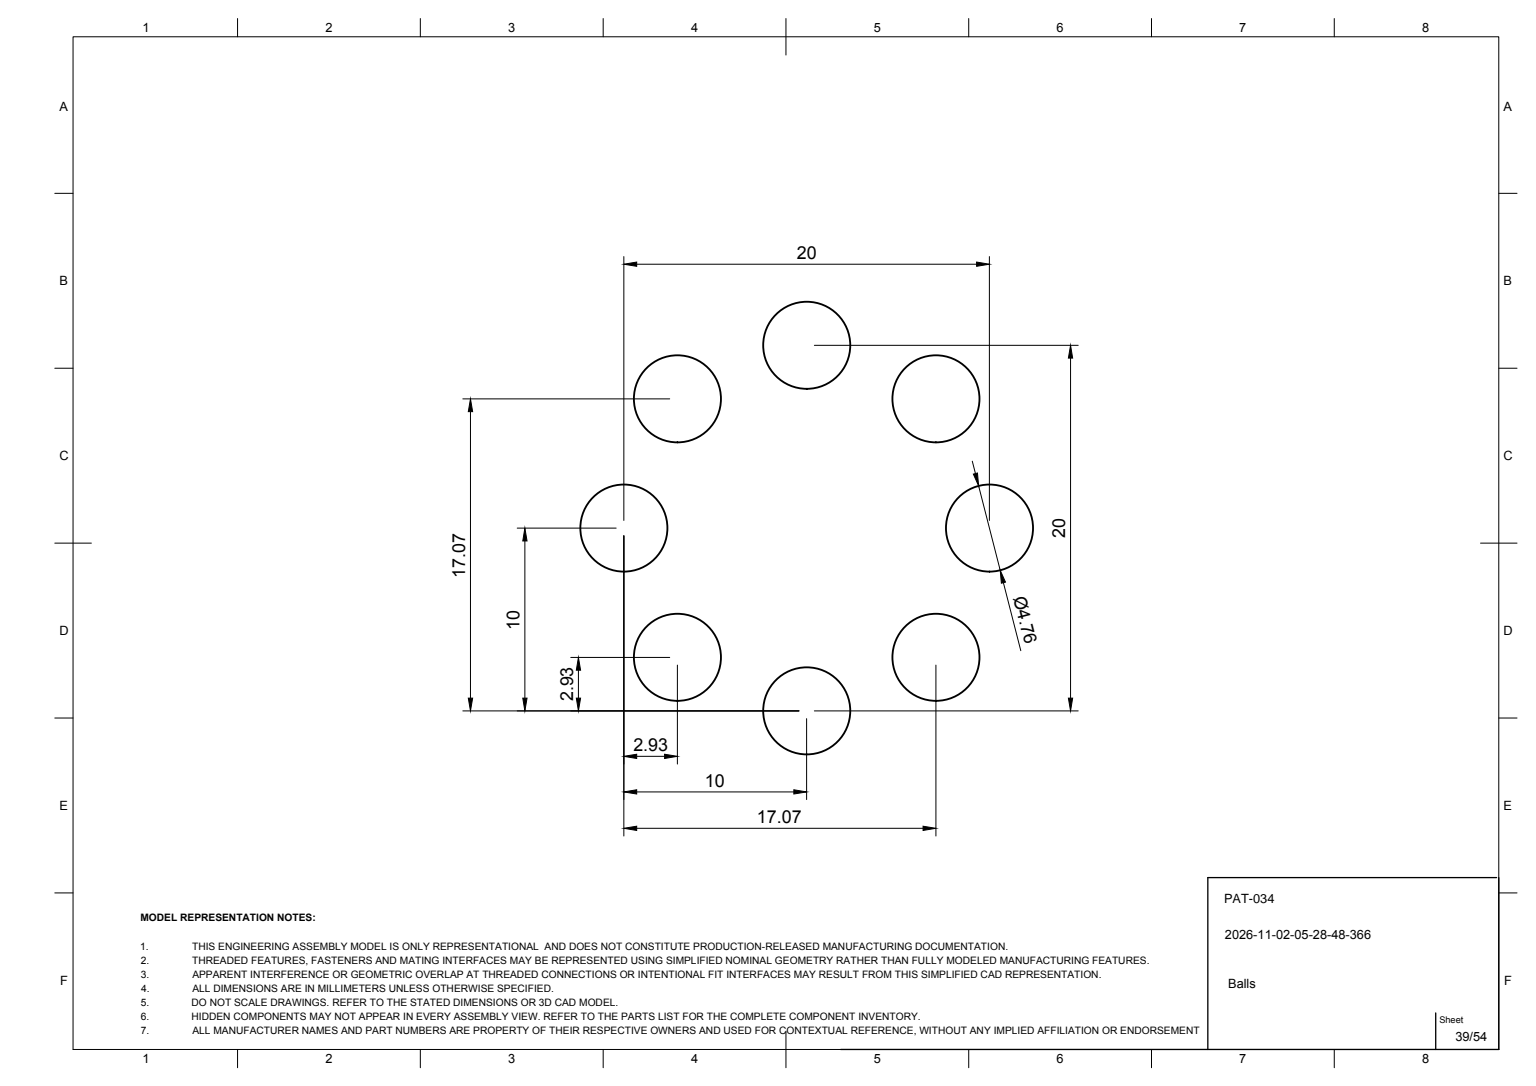
ISO-10303-21;
HEADER;
/* Generated by software containing ST-Developer
 * from STEP Tools, Inc. (www.steptools.com) 
 */

FILE_DESCRIPTION(
/* description */ ('Fatigue rig crank-slider'),
/* implementation_level */ '2;1');

FILE_NAME(
/* name */ 'Balls.step',
/* time_stamp */ '2026-10-28T03:24:50-07:00',
/* author */ (''),
/* organization */ (''),
/* preprocessor_version */ 'ST-DEVELOPER v20.2',
/* originating_system */ 'Autodesk Translation Framework v15.17.0.0',
/* authorisation */ '');

FILE_SCHEMA (('AUTOMOTIVE_DESIGN { 1 0 10303 214 3 1 1 }'));
ENDSEC;

DATA;
#10=MECHANICAL_DESIGN_GEOMETRIC_PRESENTATION_REPRESENTATION('',(#622,#623,#624,#625,#626,#627,#628,#629),#16911);
#471=SPHERICAL_SURFACE('',#10148,0.23815);
#472=SPHERICAL_SURFACE('',#10150,0.23815);
#473=SPHERICAL_SURFACE('',#10152,0.23815);
#474=SPHERICAL_SURFACE('',#10154,0.23815);
#475=SPHERICAL_SURFACE('',#10156,0.23815);
#476=SPHERICAL_SURFACE('',#10158,0.23815);
#477=SPHERICAL_SURFACE('',#10160,0.23815);
#478=SPHERICAL_SURFACE('',#10162,0.23815);
#521=SHAPE_REPRESENTATION_RELATIONSHIP('SRR','None',#17164,#571);
#571=ADVANCED_BREP_SHAPE_REPRESENTATION('',(#679,#680,#681,#682,#683,#684,
#685,#686),#16893);
#622=STYLED_ITEM('',(#17487),#679);
#623=STYLED_ITEM('',(#17487),#680);
#624=STYLED_ITEM('',(#17487),#681);
#625=STYLED_ITEM('',(#17487),#682);
#626=STYLED_ITEM('',(#17487),#683);
#627=STYLED_ITEM('',(#17487),#684);
#628=STYLED_ITEM('',(#17487),#685);
#629=STYLED_ITEM('',(#17487),#686);
#679=MANIFOLD_SOLID_BREP('Body1',#8915);
#680=MANIFOLD_SOLID_BREP('Body2',#8916);
#681=MANIFOLD_SOLID_BREP('Body3',#8917);
#682=MANIFOLD_SOLID_BREP('Body4',#8918);
#683=MANIFOLD_SOLID_BREP('Body5',#8919);
#684=MANIFOLD_SOLID_BREP('Body6',#8920);
#685=MANIFOLD_SOLID_BREP('Body7',#8921);
#686=MANIFOLD_SOLID_BREP('Body8',#8922);
#1558=FACE_OUTER_BOUND('',#2239,.T.);
#1559=FACE_OUTER_BOUND('',#2240,.T.);
#1560=FACE_OUTER_BOUND('',#2241,.T.);
#1561=FACE_OUTER_BOUND('',#2242,.T.);
#1562=FACE_OUTER_BOUND('',#2243,.T.);
#1563=FACE_OUTER_BOUND('',#2244,.T.);
#1564=FACE_OUTER_BOUND('',#2245,.T.);
#1565=FACE_OUTER_BOUND('',#2246,.T.);
#2239=EDGE_LOOP('',(#7404,#7405));
#2240=EDGE_LOOP('',(#7406,#7407));
#2241=EDGE_LOOP('',(#7408,#7409));
#2242=EDGE_LOOP('',(#7410,#7411));
#2243=EDGE_LOOP('',(#7412,#7413));
#2244=EDGE_LOOP('',(#7414,#7415));
#2245=EDGE_LOOP('',(#7416,#7417));
#2246=EDGE_LOOP('',(#7418,#7419));
#4023=CIRCLE('',#10149,0.23815);
#4024=CIRCLE('',#10151,0.23815);
#4025=CIRCLE('',#10153,0.23815);
#4026=CIRCLE('',#10155,0.23815);
#4027=CIRCLE('',#10157,0.23815);
#4028=CIRCLE('',#10159,0.23815);
#4029=CIRCLE('',#10161,0.23815);
#4030=CIRCLE('',#10163,0.23815);
#4625=VERTEX_POINT('',#15501);
#4626=VERTEX_POINT('',#15502);
#4627=VERTEX_POINT('',#15505);
#4628=VERTEX_POINT('',#15506);
#4629=VERTEX_POINT('',#15509);
#4630=VERTEX_POINT('',#15510);
#4631=VERTEX_POINT('',#15513);
#4632=VERTEX_POINT('',#15514);
#4633=VERTEX_POINT('',#15517);
#4634=VERTEX_POINT('',#15518);
#4635=VERTEX_POINT('',#15521);
#4636=VERTEX_POINT('',#15522);
#4637=VERTEX_POINT('',#15525);
#4638=VERTEX_POINT('',#15526);
#4639=VERTEX_POINT('',#15529);
#4640=VERTEX_POINT('',#15530);
#5600=EDGE_CURVE('',#4625,#4626,#4023,.T.);
#5601=EDGE_CURVE('',#4627,#4628,#4024,.T.);
#5602=EDGE_CURVE('',#4629,#4630,#4025,.T.);
#5603=EDGE_CURVE('',#4631,#4632,#4026,.T.);
#5604=EDGE_CURVE('',#4633,#4634,#4027,.T.);
#5605=EDGE_CURVE('',#4635,#4636,#4028,.T.);
#5606=EDGE_CURVE('',#4637,#4638,#4029,.T.);
#5607=EDGE_CURVE('',#4639,#4640,#4030,.T.);
#7404=ORIENTED_EDGE('',*,*,#5600,.T.);
#7405=ORIENTED_EDGE('',*,*,#5600,.F.);
#7406=ORIENTED_EDGE('',*,*,#5601,.T.);
#7407=ORIENTED_EDGE('',*,*,#5601,.F.);
#7408=ORIENTED_EDGE('',*,*,#5602,.T.);
#7409=ORIENTED_EDGE('',*,*,#5602,.F.);
#7410=ORIENTED_EDGE('',*,*,#5603,.T.);
#7411=ORIENTED_EDGE('',*,*,#5603,.F.);
#7412=ORIENTED_EDGE('',*,*,#5604,.T.);
#7413=ORIENTED_EDGE('',*,*,#5604,.F.);
#7414=ORIENTED_EDGE('',*,*,#5605,.T.);
#7415=ORIENTED_EDGE('',*,*,#5605,.F.);
#7416=ORIENTED_EDGE('',*,*,#5606,.T.);
#7417=ORIENTED_EDGE('',*,*,#5606,.F.);
#7418=ORIENTED_EDGE('',*,*,#5607,.T.);
#7419=ORIENTED_EDGE('',*,*,#5607,.F.);
#8696=ADVANCED_FACE('',(#1558),#471,.T.);
#8697=ADVANCED_FACE('',(#1559),#472,.T.);
#8698=ADVANCED_FACE('',(#1560),#473,.T.);
#8699=ADVANCED_FACE('',(#1561),#474,.T.);
#8700=ADVANCED_FACE('',(#1562),#475,.T.);
#8701=ADVANCED_FACE('',(#1563),#476,.T.);
#8702=ADVANCED_FACE('',(#1564),#477,.T.);
#8703=ADVANCED_FACE('',(#1565),#478,.T.);
#8915=CLOSED_SHELL('',(#8696));
#8916=CLOSED_SHELL('',(#8697));
#8917=CLOSED_SHELL('',(#8698));
#8918=CLOSED_SHELL('',(#8699));
#8919=CLOSED_SHELL('',(#8700));
#8920=CLOSED_SHELL('',(#8701));
#8921=CLOSED_SHELL('',(#8702));
#8922=CLOSED_SHELL('',(#8703));
#10147=AXIS2_PLACEMENT_3D('',#15499,#12271,#12272);
#10148=AXIS2_PLACEMENT_3D('',#15500,#12273,#12274);
#10149=AXIS2_PLACEMENT_3D('',#15503,#12275,#12276);
#10150=AXIS2_PLACEMENT_3D('',#15504,#12277,#12278);
#10151=AXIS2_PLACEMENT_3D('',#15507,#12279,#12280);
#10152=AXIS2_PLACEMENT_3D('',#15508,#12281,#12282);
#10153=AXIS2_PLACEMENT_3D('',#15511,#12283,#12284);
#10154=AXIS2_PLACEMENT_3D('',#15512,#12285,#12286);
#10155=AXIS2_PLACEMENT_3D('',#15515,#12287,#12288);
#10156=AXIS2_PLACEMENT_3D('',#15516,#12289,#12290);
#10157=AXIS2_PLACEMENT_3D('',#15519,#12291,#12292);
#10158=AXIS2_PLACEMENT_3D('',#15520,#12293,#12294);
#10159=AXIS2_PLACEMENT_3D('',#15523,#12295,#12296);
#10160=AXIS2_PLACEMENT_3D('',#15524,#12297,#12298);
#10161=AXIS2_PLACEMENT_3D('',#15527,#12299,#12300);
#10162=AXIS2_PLACEMENT_3D('',#15528,#12301,#12302);
#10163=AXIS2_PLACEMENT_3D('',#15531,#12303,#12304);
#12271=DIRECTION('axis',(0.,0.,1.));
#12272=DIRECTION('refdir',(1.,0.,0.));
#12273=DIRECTION('center_axis',(0.,0.,1.));
#12274=DIRECTION('ref_axis',(1.,0.,0.));
#12275=DIRECTION('center_axis',(1.22464679914735E-16,-1.,0.));
#12276=DIRECTION('ref_axis',(-1.,-1.22464679914735E-16,0.));
#12277=DIRECTION('center_axis',(0.707106781186548,0.,0.707106781186548));
#12278=DIRECTION('ref_axis',(0.707106781186548,0.,-0.707106781186548));
#12279=DIRECTION('center_axis',(8.65956056235494E-17,-1.,-8.65956056235493E-17));
#12280=DIRECTION('ref_axis',(-0.707106781186547,-1.22464679914735E-16,0.707106781186547));
#12281=DIRECTION('center_axis',(1.,0.,0.));
#12282=DIRECTION('ref_axis',(6.12323399573676E-17,0.,-1.));
#12283=DIRECTION('center_axis',(7.49879891330929E-33,-1.,-1.22464679914735E-16));
#12284=DIRECTION('ref_axis',(-6.12323399573676E-17,-1.22464679914735E-16,
1.));
#12285=DIRECTION('center_axis',(0.707106781186548,0.,-0.707106781186548));
#12286=DIRECTION('ref_axis',(-0.707106781186548,0.,-0.707106781186548));
#12287=DIRECTION('center_axis',(-8.65956056235493E-17,-1.,-8.65956056235494E-17));
#12288=DIRECTION('ref_axis',(0.707106781186547,-1.22464679914735E-16,0.707106781186547));
#12289=DIRECTION('center_axis',(0.,0.,-1.));
#12290=DIRECTION('ref_axis',(-1.,0.,-1.22464679914735E-16));
#12291=DIRECTION('center_axis',(-1.22464679914735E-16,-1.,-1.49975978266186E-32));
#12292=DIRECTION('ref_axis',(1.,-1.22464679914735E-16,1.22464679914735E-16));
#12293=DIRECTION('center_axis',(-0.707106781186547,0.,-0.707106781186548));
#12294=DIRECTION('ref_axis',(-0.707106781186548,0.,0.707106781186547));
#12295=DIRECTION('center_axis',(-8.65956056235493E-17,-1.,8.65956056235493E-17));
#12296=DIRECTION('ref_axis',(0.707106781186548,-1.22464679914735E-16,-0.707106781186547));
#12297=DIRECTION('center_axis',(-1.,0.,0.));
#12298=DIRECTION('ref_axis',(-1.83697019872103E-16,0.,1.));
#12299=DIRECTION('center_axis',(-2.24963967399279E-32,-1.,1.22464679914735E-16));
#12300=DIRECTION('ref_axis',(1.83697019872103E-16,-1.22464679914735E-16,
-1.));
#12301=DIRECTION('center_axis',(-0.707106781186548,0.,0.707106781186548));
#12302=DIRECTION('ref_axis',(0.707106781186547,0.,0.707106781186548));
#12303=DIRECTION('center_axis',(8.65956056235493E-17,-1.,8.65956056235493E-17));
#12304=DIRECTION('ref_axis',(-0.707106781186547,-1.22464679914735E-16,-0.707106781186548));
#15499=CARTESIAN_POINT('',(0.,0.,0.));
#15500=CARTESIAN_POINT('Origin',(1.,0.,0.));
#15501=CARTESIAN_POINT('',(1.,-1.78583896120461E-33,0.23815));
#15502=CARTESIAN_POINT('',(1.,-1.78583896120461E-33,-0.23815));
#15503=CARTESIAN_POINT('Origin',(1.,0.,0.));
#15504=CARTESIAN_POINT('Origin',(0.707106781186548,0.,-0.707106781186547));
#15505=CARTESIAN_POINT('',(0.875504261126124,-1.78583896120461E-33,-0.538709301246971));
#15506=CARTESIAN_POINT('',(0.538709301246971,-1.78583896120461E-33,-0.875504261126124));
#15507=CARTESIAN_POINT('Origin',(0.707106781186548,0.,-0.707106781186547));
#15508=CARTESIAN_POINT('Origin',(6.12323399573677E-17,0.,-1.));
#15509=CARTESIAN_POINT('',(0.23815,-1.78583896120461E-33,-1.));
#15510=CARTESIAN_POINT('',(-0.23815,-1.78583896120461E-33,-1.));
#15511=CARTESIAN_POINT('Origin',(6.12323399573677E-17,0.,-1.));
#15512=CARTESIAN_POINT('Origin',(-0.707106781186547,0.,-0.707106781186548));
#15513=CARTESIAN_POINT('',(-0.538709301246971,-1.78583896120461E-33,-0.875504261126124));
#15514=CARTESIAN_POINT('',(-0.875504261126124,-1.78583896120461E-33,-0.538709301246971));
#15515=CARTESIAN_POINT('Origin',(-0.707106781186547,0.,-0.707106781186548));
#15516=CARTESIAN_POINT('Origin',(-1.,0.,-1.22464679914735E-16));
#15517=CARTESIAN_POINT('',(-1.,-1.78583896120461E-33,-0.23815));
#15518=CARTESIAN_POINT('',(-1.,-1.78583896120461E-33,0.23815));
#15519=CARTESIAN_POINT('Origin',(-1.,0.,-1.22464679914735E-16));
#15520=CARTESIAN_POINT('Origin',(-0.707106781186548,0.,0.707106781186547));
#15521=CARTESIAN_POINT('',(-0.875504261126124,-7.94881478324376E-33,0.538709301246971));
#15522=CARTESIAN_POINT('',(-0.538709301246971,4.37713686083455E-33,0.875504261126124));
#15523=CARTESIAN_POINT('Origin',(-0.707106781186548,0.,0.707106781186547));
#15524=CARTESIAN_POINT('Origin',(-1.83697019872103E-16,0.,1.));
#15525=CARTESIAN_POINT('',(-0.23815,-1.78583896120461E-33,1.));
#15526=CARTESIAN_POINT('',(0.23815,-1.78583896120461E-33,1.));
#15527=CARTESIAN_POINT('Origin',(-1.83697019872103E-16,0.,1.));
#15528=CARTESIAN_POINT('Origin',(0.707106781186547,0.,0.707106781186548));
#15529=CARTESIAN_POINT('',(0.538709301246971,-4.86732687222419E-33,0.875504261126124));
#15530=CARTESIAN_POINT('',(0.875504261126124,1.29564894981497E-33,0.538709301246971));
#15531=CARTESIAN_POINT('Origin',(0.707106781186547,0.,0.707106781186548));
#16834=UNCERTAINTY_MEASURE_WITH_UNIT(LENGTH_MEASURE(0.001),#16912,
'DISTANCE_ACCURACY_VALUE',
'Maximum model space distance between geometric entities at asserted c
onnectivities');
#16852=UNCERTAINTY_MEASURE_WITH_UNIT(LENGTH_MEASURE(0.001),#16912,
'DISTANCE_ACCURACY_VALUE',
'Maximum model space distance between geometric entities at asserted c
onnectivities');
#16893=(
GEOMETRIC_REPRESENTATION_CONTEXT(3)
GLOBAL_UNCERTAINTY_ASSIGNED_CONTEXT((#16834))
GLOBAL_UNIT_ASSIGNED_CONTEXT((#16912,#16914,#16915))
REPRESENTATION_CONTEXT('','3D')
);
#16911=(
GEOMETRIC_REPRESENTATION_CONTEXT(3)
GLOBAL_UNCERTAINTY_ASSIGNED_CONTEXT((#16852))
GLOBAL_UNIT_ASSIGNED_CONTEXT((#16912,#16914,#16915))
REPRESENTATION_CONTEXT('','3D')
);
#16912=(
LENGTH_UNIT()
NAMED_UNIT(*)
SI_UNIT(.CENTI.,.METRE.)
);
#16914=(
NAMED_UNIT(*)
PLANE_ANGLE_UNIT()
SI_UNIT($,.RADIAN.)
);
#16915=(
NAMED_UNIT(*)
SI_UNIT($,.STERADIAN.)
SOLID_ANGLE_UNIT()
);
#16956=SHAPE_DEFINITION_REPRESENTATION(#17016,#17164);
#17016=PRODUCT_DEFINITION_SHAPE('',$,#17223);
#17164=SHAPE_REPRESENTATION('',(#10147),#16893);
#17182=PRODUCT_DEFINITION_CONTEXT('part definition',#17358,'design');
#17223=PRODUCT_DEFINITION('Balls','Balls',#17281,#17182);
#17281=PRODUCT_DEFINITION_FORMATION('',$,#17400);
#17358=APPLICATION_CONTEXT(
'Core Data for Automotive Mechanical Design Process');
#17359=PRODUCT_CONTEXT('part definition',#17358,'mechanical');
#17400=PRODUCT('Balls','Balls','Balls',(#17359));
#17481=COLOUR_RGB('Grey',0.48,0.52,0.57);
#17482=FILL_AREA_STYLE_COLOUR('',#17481);
#17483=FILL_AREA_STYLE('',(#17482));
#17484=SURFACE_STYLE_FILL_AREA(#17483);
#17485=SURFACE_SIDE_STYLE('',(#17484));
#17486=SURFACE_STYLE_USAGE(.BOTH.,#17485);
#17487=PRESENTATION_STYLE_ASSIGNMENT((#17486));
ENDSEC;
END-ISO-10303-21;
